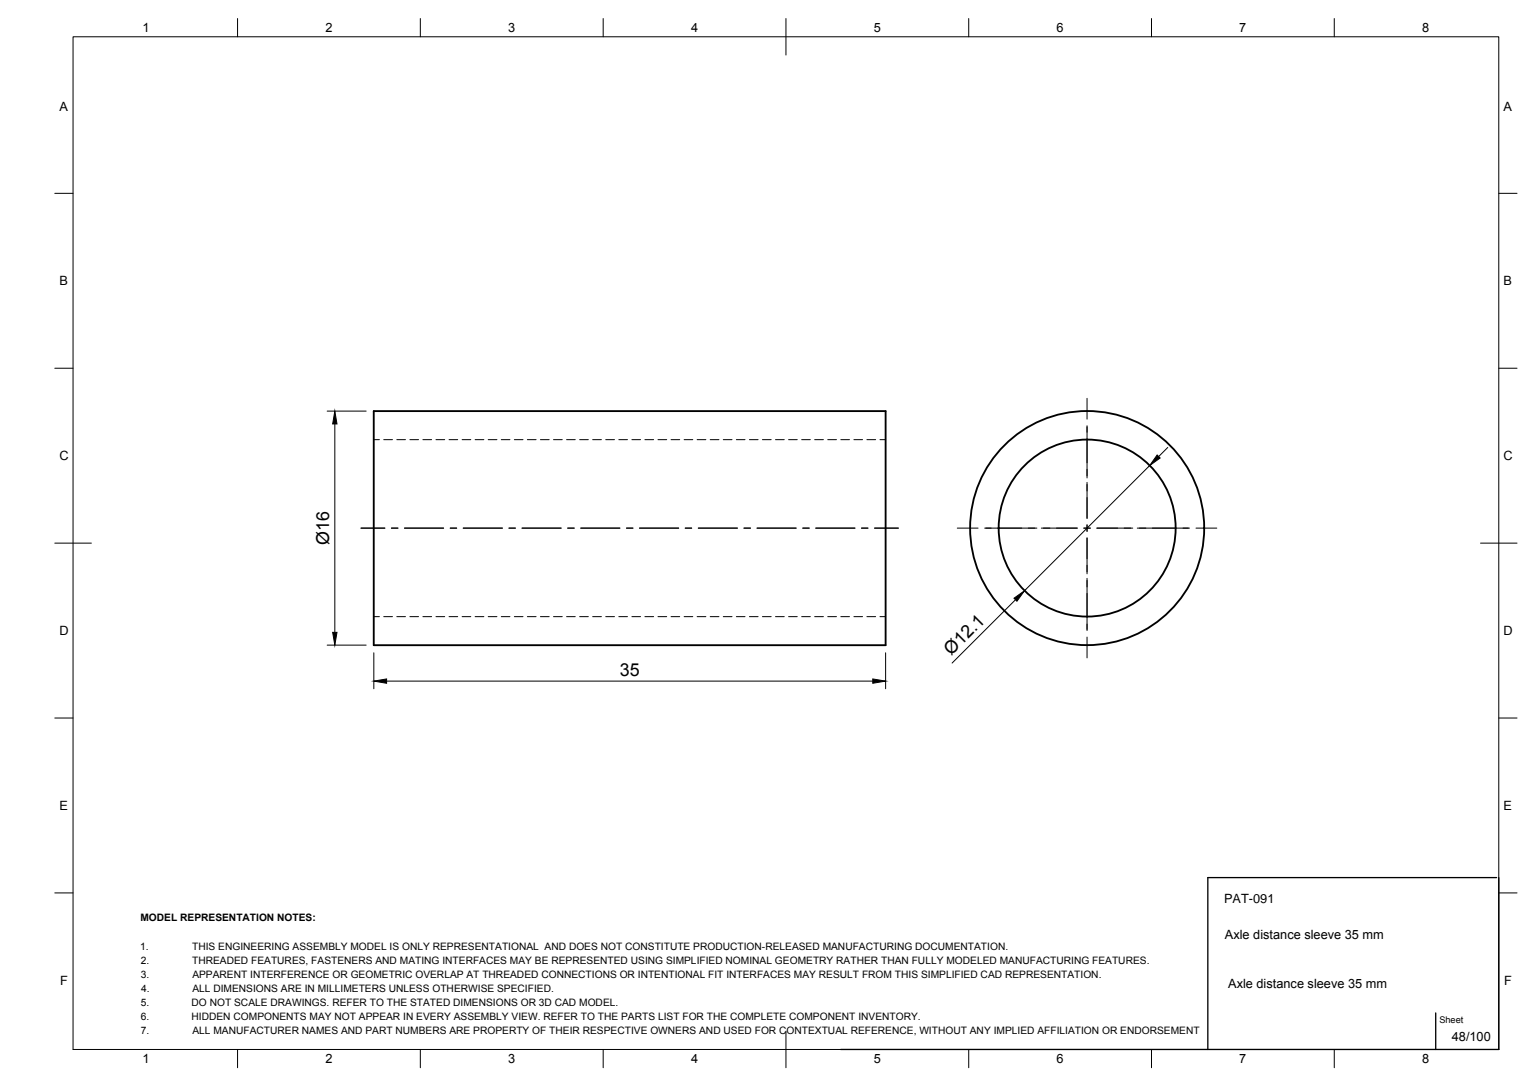
ISO-10303-21;
HEADER;
/* Generated by software containing ST-Developer
 * from STEP Tools, Inc. (www.steptools.com) 
 */

FILE_DESCRIPTION(
/* description */ ('PAT-091'),
/* implementation_level */ '2;1');

FILE_NAME(
/* name */ 'Axle distance sleeve 35 mm.step',
/* time_stamp */ '2026-10-27T15:34:44-07:00',
/* author */ (''),
/* organization */ (''),
/* preprocessor_version */ 'ST-DEVELOPER v20.2',
/* originating_system */ 'Autodesk Translation Framework v15.17.0.0',
/* authorisation */ '');

FILE_SCHEMA (('AUTOMOTIVE_DESIGN { 1 0 10303 214 3 1 1 }'));
ENDSEC;

DATA;
#10=MECHANICAL_DESIGN_GEOMETRIC_PRESENTATION_REPRESENTATION('',(#1011),#25100);
#791=SHAPE_REPRESENTATION_RELATIONSHIP('SRR','None',#25554,#901);
#901=ADVANCED_BREP_SHAPE_REPRESENTATION('',(#1133),#25024);
#1011=STYLED_ITEM('',(#26191),#1133);
#1133=MANIFOLD_SOLID_BREP('Body1',#13290);
#1428=FACE_BOUND('',#3425,.T.);
#1429=FACE_BOUND('',#3427,.T.);
#1819=PLANE('',#15257);
#1820=PLANE('',#15258);
#2391=FACE_OUTER_BOUND('',#3422,.T.);
#2392=FACE_OUTER_BOUND('',#3423,.T.);
#2393=FACE_OUTER_BOUND('',#3424,.T.);
#2394=FACE_OUTER_BOUND('',#3426,.T.);
#3422=EDGE_LOOP('',(#10320,#10321,#10322,#10323));
#3423=EDGE_LOOP('',(#10324,#10325,#10326,#10327));
#3424=EDGE_LOOP('',(#10328));
#3425=EDGE_LOOP('',(#10329));
#3426=EDGE_LOOP('',(#10330));
#3427=EDGE_LOOP('',(#10331));
#4503=LINE('',#22498,#5243);
#4504=LINE('',#22504,#5244);
#5243=VECTOR('',#18183,0.604999999999997);
#5244=VECTOR('',#18190,0.799999999999997);
#5897=CIRCLE('',#15252,0.604999999999997);
#5898=CIRCLE('',#15253,0.604999999999997);
#5899=CIRCLE('',#15255,0.799999999999997);
#5900=CIRCLE('',#15256,0.799999999999997);
#6830=VERTEX_POINT('',#22495);
#6831=VERTEX_POINT('',#22497);
#6832=VERTEX_POINT('',#22501);
#6833=VERTEX_POINT('',#22503);
#8095=EDGE_CURVE('',#6830,#6830,#5897,.T.);
#8096=EDGE_CURVE('',#6830,#6831,#4503,.T.);
#8097=EDGE_CURVE('',#6831,#6831,#5898,.T.);
#8098=EDGE_CURVE('',#6832,#6832,#5899,.T.);
#8099=EDGE_CURVE('',#6832,#6833,#4504,.T.);
#8100=EDGE_CURVE('',#6833,#6833,#5900,.T.);
#10320=ORIENTED_EDGE('',*,*,#8095,.F.);
#10321=ORIENTED_EDGE('',*,*,#8096,.T.);
#10322=ORIENTED_EDGE('',*,*,#8097,.T.);
#10323=ORIENTED_EDGE('',*,*,#8096,.F.);
#10324=ORIENTED_EDGE('',*,*,#8098,.F.);
#10325=ORIENTED_EDGE('',*,*,#8099,.T.);
#10326=ORIENTED_EDGE('',*,*,#8100,.T.);
#10327=ORIENTED_EDGE('',*,*,#8099,.F.);
#10328=ORIENTED_EDGE('',*,*,#8098,.T.);
#10329=ORIENTED_EDGE('',*,*,#8095,.T.);
#10330=ORIENTED_EDGE('',*,*,#8100,.F.);
#10331=ORIENTED_EDGE('',*,*,#8097,.F.);
#12216=CYLINDRICAL_SURFACE('',#15251,0.604999999999997);
#12217=CYLINDRICAL_SURFACE('',#15254,0.799999999999997);
#12758=ADVANCED_FACE('',(#2391),#12216,.F.);
#12759=ADVANCED_FACE('',(#2392),#12217,.T.);
#12760=ADVANCED_FACE('',(#2393,#1428),#1819,.T.);
#12761=ADVANCED_FACE('',(#2394,#1429),#1820,.F.);
#13290=CLOSED_SHELL('',(#12758,#12759,#12760,#12761));
#15250=AXIS2_PLACEMENT_3D('',#22493,#18177,#18178);
#15251=AXIS2_PLACEMENT_3D('',#22494,#18179,#18180);
#15252=AXIS2_PLACEMENT_3D('',#22496,#18181,#18182);
#15253=AXIS2_PLACEMENT_3D('',#22499,#18184,#18185);
#15254=AXIS2_PLACEMENT_3D('',#22500,#18186,#18187);
#15255=AXIS2_PLACEMENT_3D('',#22502,#18188,#18189);
#15256=AXIS2_PLACEMENT_3D('',#22505,#18191,#18192);
#15257=AXIS2_PLACEMENT_3D('',#22506,#18193,#18194);
#15258=AXIS2_PLACEMENT_3D('',#22507,#18195,#18196);
#18177=DIRECTION('axis',(0.,0.,1.));
#18178=DIRECTION('refdir',(1.,0.,0.));
#18179=DIRECTION('center_axis',(0.,1.,0.));
#18180=DIRECTION('ref_axis',(1.,0.,0.));
#18181=DIRECTION('center_axis',(0.,-1.,0.));
#18182=DIRECTION('ref_axis',(1.,0.,0.));
#18183=DIRECTION('',(0.,-1.,0.));
#18184=DIRECTION('center_axis',(0.,-1.,0.));
#18185=DIRECTION('ref_axis',(1.,0.,0.));
#18186=DIRECTION('center_axis',(0.,1.,0.));
#18187=DIRECTION('ref_axis',(1.,0.,0.));
#18188=DIRECTION('center_axis',(0.,1.,0.));
#18189=DIRECTION('ref_axis',(1.,0.,0.));
#18190=DIRECTION('',(0.,-1.,0.));
#18191=DIRECTION('center_axis',(0.,1.,0.));
#18192=DIRECTION('ref_axis',(1.,0.,0.));
#18193=DIRECTION('center_axis',(0.,1.,0.));
#18194=DIRECTION('ref_axis',(1.,0.,0.));
#18195=DIRECTION('center_axis',(0.,1.,0.));
#18196=DIRECTION('ref_axis',(1.,0.,0.));
#22493=CARTESIAN_POINT('',(0.,0.,0.));
#22494=CARTESIAN_POINT('Origin',(38.7298334620742,3.5,3.));
#22495=CARTESIAN_POINT('',(38.1248334620742,7.,3.));
#22496=CARTESIAN_POINT('Origin',(38.7298334620742,7.,3.));
#22497=CARTESIAN_POINT('',(38.1248334620742,3.5,3.));
#22498=CARTESIAN_POINT('',(38.1248334620742,3.5,3.));
#22499=CARTESIAN_POINT('Origin',(38.7298334620742,3.5,3.));
#22500=CARTESIAN_POINT('Origin',(38.7298334620742,3.5,3.));
#22501=CARTESIAN_POINT('',(37.9298334620742,7.,3.));
#22502=CARTESIAN_POINT('Origin',(38.7298334620742,7.,3.));
#22503=CARTESIAN_POINT('',(37.9298334620742,3.5,3.));
#22504=CARTESIAN_POINT('',(37.9298334620742,3.5,3.));
#22505=CARTESIAN_POINT('Origin',(38.7298334620742,3.5,3.));
#22506=CARTESIAN_POINT('Origin',(38.7298334620742,7.,3.));
#22507=CARTESIAN_POINT('Origin',(38.7298334620742,3.5,3.));
#24903=UNCERTAINTY_MEASURE_WITH_UNIT(LENGTH_MEASURE(0.001),#25101,
'DISTANCE_ACCURACY_VALUE',
'Maximum model space distance between geometric entities at asserted c
onnectivities');
#24979=UNCERTAINTY_MEASURE_WITH_UNIT(LENGTH_MEASURE(0.001),#25101,
'DISTANCE_ACCURACY_VALUE',
'Maximum model space distance between geometric entities at asserted c
onnectivities');
#25024=(
GEOMETRIC_REPRESENTATION_CONTEXT(3)
GLOBAL_UNCERTAINTY_ASSIGNED_CONTEXT((#24903))
GLOBAL_UNIT_ASSIGNED_CONTEXT((#25101,#25103,#25104))
REPRESENTATION_CONTEXT('','3D')
);
#25100=(
GEOMETRIC_REPRESENTATION_CONTEXT(3)
GLOBAL_UNCERTAINTY_ASSIGNED_CONTEXT((#24979))
GLOBAL_UNIT_ASSIGNED_CONTEXT((#25101,#25103,#25104))
REPRESENTATION_CONTEXT('','3D')
);
#25101=(
LENGTH_UNIT()
NAMED_UNIT(*)
SI_UNIT(.CENTI.,.METRE.)
);
#25103=(
NAMED_UNIT(*)
PLANE_ANGLE_UNIT()
SI_UNIT($,.RADIAN.)
);
#25104=(
NAMED_UNIT(*)
SI_UNIT($,.STERADIAN.)
SOLID_ANGLE_UNIT()
);
#25149=SHAPE_DEFINITION_REPRESENTATION(#25269,#25554);
#25269=PRODUCT_DEFINITION_SHAPE('',$,#25675);
#25554=SHAPE_REPRESENTATION('',(#15250),#25024);
#25630=PRODUCT_DEFINITION_CONTEXT('part definition',#25992,'design');
#25675=PRODUCT_DEFINITION('Axle distance sleeve 35 mm',
'Axle distance sleeve 35 mm',#25795,#25630);
#25795=PRODUCT_DEFINITION_FORMATION('',$,#26038);
#25992=APPLICATION_CONTEXT(
'Core Data for Automotive Mechanical Design Process');
#25993=PRODUCT_CONTEXT('part definition',#25992,'mechanical');
#26038=PRODUCT('Axle distance sleeve 35 mm',
'Axle distance sleeve 35 mm','Axle distance sleeve 35 mm',(#25993));
#26185=COLOUR_RGB('Grey',0.48,0.52,0.57);
#26186=FILL_AREA_STYLE_COLOUR('',#26185);
#26187=FILL_AREA_STYLE('',(#26186));
#26188=SURFACE_STYLE_FILL_AREA(#26187);
#26189=SURFACE_SIDE_STYLE('',(#26188));
#26190=SURFACE_STYLE_USAGE(.BOTH.,#26189);
#26191=PRESENTATION_STYLE_ASSIGNMENT((#26190));
ENDSEC;
END-ISO-10303-21;
